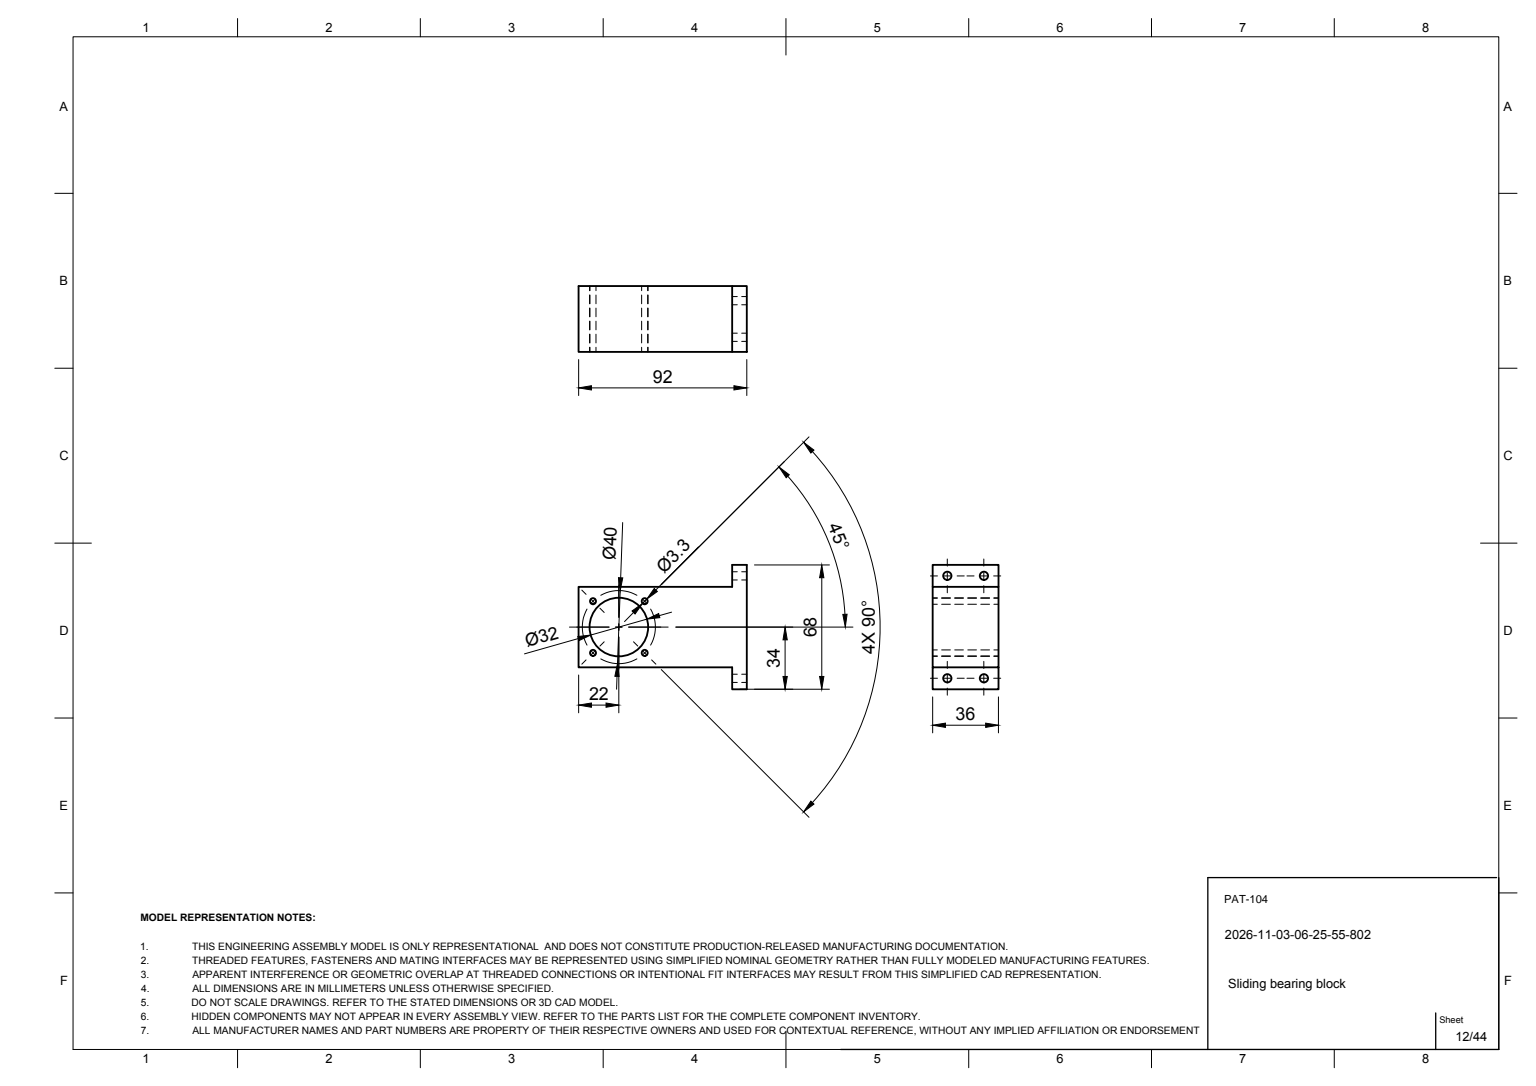
ISO-10303-21;
HEADER;
/* Generated by software containing ST-Developer
 * from STEP Tools, Inc. (www.steptools.com) 
 */

FILE_DESCRIPTION(
/* description */ ('Timing belt drive module 2 mm Pitch Timing 20T-40T'),

/* implementation_level */ '2;1');

FILE_NAME(
/* name */ 'Sliding bearing block.step',
/* time_stamp */ '2026-10-28T03:25:12-07:00',
/* author */ (''),
/* organization */ (''),
/* preprocessor_version */ 'ST-DEVELOPER v20.2',
/* originating_system */ 'Autodesk Translation Framework v15.17.0.0',
/* authorisation */ '');

FILE_SCHEMA (('AUTOMOTIVE_DESIGN { 1 0 10303 214 3 1 1 }'));
ENDSEC;

DATA;
#10=MECHANICAL_DESIGN_GEOMETRIC_PRESENTATION_REPRESENTATION('',(#531),#17830);
#445=SHAPE_REPRESENTATION_RELATIONSHIP('SRR','None',#18015,#488);
#488=ADVANCED_BREP_SHAPE_REPRESENTATION('',(#589),#17790);
#531=STYLED_ITEM('',(#18317),#589);
#589=MANIFOLD_SOLID_BREP('Body1',#8988);
#673=FACE_BOUND('',#1620,.T.);
#674=FACE_BOUND('',#1621,.T.);
#675=FACE_BOUND('',#1623,.T.);
#676=FACE_BOUND('',#1624,.T.);
#677=FACE_BOUND('',#1628,.T.);
#678=FACE_BOUND('',#1629,.T.);
#679=FACE_BOUND('',#1630,.T.);
#680=FACE_BOUND('',#1631,.T.);
#681=FACE_BOUND('',#1632,.T.);
#682=FACE_BOUND('',#1635,.T.);
#683=FACE_BOUND('',#1636,.T.);
#684=FACE_BOUND('',#1637,.T.);
#685=FACE_BOUND('',#1638,.T.);
#686=FACE_BOUND('',#1639,.T.);
#687=FACE_BOUND('',#1643,.T.);
#688=FACE_BOUND('',#1644,.T.);
#689=FACE_BOUND('',#1645,.T.);
#690=FACE_BOUND('',#1646,.T.);
#821=PLANE('',#9734);
#822=PLANE('',#9735);
#823=PLANE('',#9736);
#824=PLANE('',#9737);
#825=PLANE('',#9738);
#826=PLANE('',#9739);
#827=PLANE('',#9740);
#828=PLANE('',#9741);
#829=PLANE('',#9742);
#830=PLANE('',#9743);
#1053=FACE_OUTER_BOUND('',#1610,.T.);
#1054=FACE_OUTER_BOUND('',#1611,.T.);
#1055=FACE_OUTER_BOUND('',#1612,.T.);
#1056=FACE_OUTER_BOUND('',#1613,.T.);
#1057=FACE_OUTER_BOUND('',#1614,.T.);
#1058=FACE_OUTER_BOUND('',#1615,.T.);
#1059=FACE_OUTER_BOUND('',#1616,.T.);
#1060=FACE_OUTER_BOUND('',#1617,.T.);
#1061=FACE_OUTER_BOUND('',#1618,.T.);
#1062=FACE_OUTER_BOUND('',#1619,.T.);
#1063=FACE_OUTER_BOUND('',#1622,.T.);
#1064=FACE_OUTER_BOUND('',#1625,.T.);
#1065=FACE_OUTER_BOUND('',#1626,.T.);
#1066=FACE_OUTER_BOUND('',#1627,.T.);
#1067=FACE_OUTER_BOUND('',#1633,.T.);
#1068=FACE_OUTER_BOUND('',#1634,.T.);
#1069=FACE_OUTER_BOUND('',#1640,.T.);
#1070=FACE_OUTER_BOUND('',#1641,.T.);
#1071=FACE_OUTER_BOUND('',#1642,.T.);
#1610=EDGE_LOOP('',(#6211,#6212,#6213,#6214));
#1611=EDGE_LOOP('',(#6215,#6216,#6217,#6218));
#1612=EDGE_LOOP('',(#6219,#6220,#6221,#6222));
#1613=EDGE_LOOP('',(#6223,#6224,#6225,#6226));
#1614=EDGE_LOOP('',(#6227,#6228,#6229,#6230));
#1615=EDGE_LOOP('',(#6231,#6232,#6233,#6234));
#1616=EDGE_LOOP('',(#6235,#6236,#6237,#6238));
#1617=EDGE_LOOP('',(#6239,#6240,#6241,#6242));
#1618=EDGE_LOOP('',(#6243,#6244,#6245,#6246));
#1619=EDGE_LOOP('',(#6247,#6248,#6249,#6250));
#1620=EDGE_LOOP('',(#6251));
#1621=EDGE_LOOP('',(#6252));
#1622=EDGE_LOOP('',(#6253,#6254,#6255,#6256));
#1623=EDGE_LOOP('',(#6257));
#1624=EDGE_LOOP('',(#6258));
#1625=EDGE_LOOP('',(#6259,#6260,#6261,#6262));
#1626=EDGE_LOOP('',(#6263,#6264,#6265,#6266));
#1627=EDGE_LOOP('',(#6267,#6268,#6269,#6270,#6271,#6272,#6273,#6274));
#1628=EDGE_LOOP('',(#6275));
#1629=EDGE_LOOP('',(#6276));
#1630=EDGE_LOOP('',(#6277));
#1631=EDGE_LOOP('',(#6278));
#1632=EDGE_LOOP('',(#6279));
#1633=EDGE_LOOP('',(#6280,#6281,#6282,#6283));
#1634=EDGE_LOOP('',(#6284,#6285,#6286,#6287,#6288,#6289,#6290,#6291));
#1635=EDGE_LOOP('',(#6292));
#1636=EDGE_LOOP('',(#6293));
#1637=EDGE_LOOP('',(#6294));
#1638=EDGE_LOOP('',(#6295));
#1639=EDGE_LOOP('',(#6296));
#1640=EDGE_LOOP('',(#6297,#6298,#6299,#6300));
#1641=EDGE_LOOP('',(#6301,#6302,#6303,#6304));
#1642=EDGE_LOOP('',(#6305,#6306,#6307,#6308));
#1643=EDGE_LOOP('',(#6309));
#1644=EDGE_LOOP('',(#6310));
#1645=EDGE_LOOP('',(#6311));
#1646=EDGE_LOOP('',(#6312));
#2230=CIRCLE('',#9708,0.165);
#2231=CIRCLE('',#9709,0.165);
#2232=CIRCLE('',#9711,0.165);
#2233=CIRCLE('',#9712,0.165);
#2234=CIRCLE('',#9714,0.164999999999999);
#2235=CIRCLE('',#9715,0.164999999999999);
#2236=CIRCLE('',#9717,0.164999999999999);
#2237=CIRCLE('',#9718,0.164999999999999);
#2238=CIRCLE('',#9720,1.6);
#2239=CIRCLE('',#9721,1.6);
#2240=CIRCLE('',#9723,0.225);
#2241=CIRCLE('',#9724,0.225);
#2242=CIRCLE('',#9726,0.225);
#2243=CIRCLE('',#9727,0.225);
#2244=CIRCLE('',#9729,0.225);
#2245=CIRCLE('',#9730,0.225);
#2246=CIRCLE('',#9732,0.225);
#2247=CIRCLE('',#9733,0.225);
#2919=LINE('',#14343,#3397);
#2920=LINE('',#14349,#3398);
#2921=LINE('',#14355,#3399);
#2922=LINE('',#14361,#3400);
#2923=LINE('',#14367,#3401);
#2924=LINE('',#14373,#3402);
#2925=LINE('',#14379,#3403);
#2926=LINE('',#14385,#3404);
#2927=LINE('',#14391,#3405);
#2928=LINE('',#14396,#3406);
#2929=LINE('',#14398,#3407);
#2930=LINE('',#14400,#3408);
#2931=LINE('',#14401,#3409);
#2932=LINE('',#14405,#3410);
#2933=LINE('',#14407,#3411);
#2934=LINE('',#14409,#3412);
#2935=LINE('',#14410,#3413);
#2936=LINE('',#14413,#3414);
#2937=LINE('',#14415,#3415);
#2938=LINE('',#14416,#3416);
#2939=LINE('',#14419,#3417);
#2940=LINE('',#14421,#3418);
#2941=LINE('',#14422,#3419);
#2942=LINE('',#14425,#3420);
#2943=LINE('',#14427,#3421);
#2944=LINE('',#14428,#3422);
#2945=LINE('',#14429,#3423);
#2946=LINE('',#14432,#3424);
#2947=LINE('',#14433,#3425);
#2948=LINE('',#14436,#3426);
#2949=LINE('',#14437,#3427);
#2950=LINE('',#14438,#3428);
#2951=LINE('',#14440,#3429);
#3397=VECTOR('',#11324,0.165);
#3398=VECTOR('',#11331,0.165);
#3399=VECTOR('',#11338,0.164999999999999);
#3400=VECTOR('',#11345,0.164999999999999);
#3401=VECTOR('',#11352,1.6);
#3402=VECTOR('',#11359,0.225);
#3403=VECTOR('',#11366,0.225);
#3404=VECTOR('',#11373,0.225);
#3405=VECTOR('',#11380,0.225);
#3406=VECTOR('',#11385,1.);
#3407=VECTOR('',#11386,1.);
#3408=VECTOR('',#11387,1.);
#3409=VECTOR('',#11388,1.);
#3410=VECTOR('',#11391,1.);
#3411=VECTOR('',#11392,1.);
#3412=VECTOR('',#11393,1.);
#3413=VECTOR('',#11394,1.);
#3414=VECTOR('',#11397,1.);
#3415=VECTOR('',#11398,1.);
#3416=VECTOR('',#11399,1.);
#3417=VECTOR('',#11402,1.);
#3418=VECTOR('',#11403,1.);
#3419=VECTOR('',#11404,1.);
#3420=VECTOR('',#11407,1.);
#3421=VECTOR('',#11408,1.);
#3422=VECTOR('',#11409,1.);
#3423=VECTOR('',#11410,1.);
#3424=VECTOR('',#11413,1.);
#3425=VECTOR('',#11414,1.);
#3426=VECTOR('',#11417,1.);
#3427=VECTOR('',#11418,1.);
#3428=VECTOR('',#11419,1.);
#3429=VECTOR('',#11422,1.);
#3892=VERTEX_POINT('',#14340);
#3893=VERTEX_POINT('',#14342);
#3894=VERTEX_POINT('',#14346);
#3895=VERTEX_POINT('',#14348);
#3896=VERTEX_POINT('',#14352);
#3897=VERTEX_POINT('',#14354);
#3898=VERTEX_POINT('',#14358);
#3899=VERTEX_POINT('',#14360);
#3900=VERTEX_POINT('',#14364);
#3901=VERTEX_POINT('',#14366);
#3902=VERTEX_POINT('',#14370);
#3903=VERTEX_POINT('',#14372);
#3904=VERTEX_POINT('',#14376);
#3905=VERTEX_POINT('',#14378);
#3906=VERTEX_POINT('',#14382);
#3907=VERTEX_POINT('',#14384);
#3908=VERTEX_POINT('',#14388);
#3909=VERTEX_POINT('',#14390);
#3910=VERTEX_POINT('',#14394);
#3911=VERTEX_POINT('',#14395);
#3912=VERTEX_POINT('',#14397);
#3913=VERTEX_POINT('',#14399);
#3914=VERTEX_POINT('',#14403);
#3915=VERTEX_POINT('',#14404);
#3916=VERTEX_POINT('',#14406);
#3917=VERTEX_POINT('',#14408);
#3918=VERTEX_POINT('',#14412);
#3919=VERTEX_POINT('',#14414);
#3920=VERTEX_POINT('',#14418);
#3921=VERTEX_POINT('',#14420);
#3922=VERTEX_POINT('',#14424);
#3923=VERTEX_POINT('',#14426);
#3924=VERTEX_POINT('',#14431);
#3925=VERTEX_POINT('',#14435);
#4788=EDGE_CURVE('',#3892,#3892,#2230,.T.);
#4789=EDGE_CURVE('',#3892,#3893,#2919,.T.);
#4790=EDGE_CURVE('',#3893,#3893,#2231,.T.);
#4791=EDGE_CURVE('',#3894,#3894,#2232,.T.);
#4792=EDGE_CURVE('',#3894,#3895,#2920,.T.);
#4793=EDGE_CURVE('',#3895,#3895,#2233,.T.);
#4794=EDGE_CURVE('',#3896,#3896,#2234,.T.);
#4795=EDGE_CURVE('',#3896,#3897,#2921,.T.);
#4796=EDGE_CURVE('',#3897,#3897,#2235,.T.);
#4797=EDGE_CURVE('',#3898,#3898,#2236,.T.);
#4798=EDGE_CURVE('',#3898,#3899,#2922,.T.);
#4799=EDGE_CURVE('',#3899,#3899,#2237,.T.);
#4800=EDGE_CURVE('',#3900,#3900,#2238,.T.);
#4801=EDGE_CURVE('',#3900,#3901,#2923,.T.);
#4802=EDGE_CURVE('',#3901,#3901,#2239,.T.);
#4803=EDGE_CURVE('',#3902,#3902,#2240,.T.);
#4804=EDGE_CURVE('',#3902,#3903,#2924,.T.);
#4805=EDGE_CURVE('',#3903,#3903,#2241,.T.);
#4806=EDGE_CURVE('',#3904,#3904,#2242,.T.);
#4807=EDGE_CURVE('',#3904,#3905,#2925,.T.);
#4808=EDGE_CURVE('',#3905,#3905,#2243,.T.);
#4809=EDGE_CURVE('',#3906,#3906,#2244,.T.);
#4810=EDGE_CURVE('',#3906,#3907,#2926,.T.);
#4811=EDGE_CURVE('',#3907,#3907,#2245,.T.);
#4812=EDGE_CURVE('',#3908,#3908,#2246,.T.);
#4813=EDGE_CURVE('',#3908,#3909,#2927,.T.);
#4814=EDGE_CURVE('',#3909,#3909,#2247,.T.);
#4815=EDGE_CURVE('',#3910,#3911,#2928,.T.);
#4816=EDGE_CURVE('',#3912,#3910,#2929,.T.);
#4817=EDGE_CURVE('',#3912,#3913,#2930,.T.);
#4818=EDGE_CURVE('',#3911,#3913,#2931,.T.);
#4819=EDGE_CURVE('',#3914,#3915,#2932,.T.);
#4820=EDGE_CURVE('',#3916,#3914,#2933,.T.);
#4821=EDGE_CURVE('',#3917,#3916,#2934,.T.);
#4822=EDGE_CURVE('',#3915,#3917,#2935,.T.);
#4823=EDGE_CURVE('',#3917,#3918,#2936,.T.);
#4824=EDGE_CURVE('',#3919,#3916,#2937,.T.);
#4825=EDGE_CURVE('',#3918,#3919,#2938,.T.);
#4826=EDGE_CURVE('',#3920,#3912,#2939,.T.);
#4827=EDGE_CURVE('',#3920,#3921,#2940,.T.);
#4828=EDGE_CURVE('',#3913,#3921,#2941,.T.);
#4829=EDGE_CURVE('',#3910,#3922,#2942,.T.);
#4830=EDGE_CURVE('',#3923,#3922,#2943,.T.);
#4831=EDGE_CURVE('',#3915,#3923,#2944,.T.);
#4832=EDGE_CURVE('',#3918,#3920,#2945,.T.);
#4833=EDGE_CURVE('',#3911,#3924,#2946,.T.);
#4834=EDGE_CURVE('',#3922,#3924,#2947,.T.);
#4835=EDGE_CURVE('',#3914,#3925,#2948,.T.);
#4836=EDGE_CURVE('',#3924,#3925,#2949,.T.);
#4837=EDGE_CURVE('',#3921,#3919,#2950,.T.);
#4838=EDGE_CURVE('',#3925,#3923,#2951,.T.);
#6211=ORIENTED_EDGE('',*,*,#4788,.F.);
#6212=ORIENTED_EDGE('',*,*,#4789,.T.);
#6213=ORIENTED_EDGE('',*,*,#4790,.F.);
#6214=ORIENTED_EDGE('',*,*,#4789,.F.);
#6215=ORIENTED_EDGE('',*,*,#4791,.F.);
#6216=ORIENTED_EDGE('',*,*,#4792,.T.);
#6217=ORIENTED_EDGE('',*,*,#4793,.F.);
#6218=ORIENTED_EDGE('',*,*,#4792,.F.);
#6219=ORIENTED_EDGE('',*,*,#4794,.F.);
#6220=ORIENTED_EDGE('',*,*,#4795,.T.);
#6221=ORIENTED_EDGE('',*,*,#4796,.F.);
#6222=ORIENTED_EDGE('',*,*,#4795,.F.);
#6223=ORIENTED_EDGE('',*,*,#4797,.F.);
#6224=ORIENTED_EDGE('',*,*,#4798,.T.);
#6225=ORIENTED_EDGE('',*,*,#4799,.F.);
#6226=ORIENTED_EDGE('',*,*,#4798,.F.);
#6227=ORIENTED_EDGE('',*,*,#4800,.F.);
#6228=ORIENTED_EDGE('',*,*,#4801,.T.);
#6229=ORIENTED_EDGE('',*,*,#4802,.F.);
#6230=ORIENTED_EDGE('',*,*,#4801,.F.);
#6231=ORIENTED_EDGE('',*,*,#4803,.F.);
#6232=ORIENTED_EDGE('',*,*,#4804,.T.);
#6233=ORIENTED_EDGE('',*,*,#4805,.F.);
#6234=ORIENTED_EDGE('',*,*,#4804,.F.);
#6235=ORIENTED_EDGE('',*,*,#4806,.F.);
#6236=ORIENTED_EDGE('',*,*,#4807,.T.);
#6237=ORIENTED_EDGE('',*,*,#4808,.F.);
#6238=ORIENTED_EDGE('',*,*,#4807,.F.);
#6239=ORIENTED_EDGE('',*,*,#4809,.F.);
#6240=ORIENTED_EDGE('',*,*,#4810,.T.);
#6241=ORIENTED_EDGE('',*,*,#4811,.F.);
#6242=ORIENTED_EDGE('',*,*,#4810,.F.);
#6243=ORIENTED_EDGE('',*,*,#4812,.F.);
#6244=ORIENTED_EDGE('',*,*,#4813,.T.);
#6245=ORIENTED_EDGE('',*,*,#4814,.F.);
#6246=ORIENTED_EDGE('',*,*,#4813,.F.);
#6247=ORIENTED_EDGE('',*,*,#4815,.F.);
#6248=ORIENTED_EDGE('',*,*,#4816,.F.);
#6249=ORIENTED_EDGE('',*,*,#4817,.T.);
#6250=ORIENTED_EDGE('',*,*,#4818,.F.);
#6251=ORIENTED_EDGE('',*,*,#4805,.T.);
#6252=ORIENTED_EDGE('',*,*,#4814,.T.);
#6253=ORIENTED_EDGE('',*,*,#4819,.F.);
#6254=ORIENTED_EDGE('',*,*,#4820,.F.);
#6255=ORIENTED_EDGE('',*,*,#4821,.F.);
#6256=ORIENTED_EDGE('',*,*,#4822,.F.);
#6257=ORIENTED_EDGE('',*,*,#4808,.T.);
#6258=ORIENTED_EDGE('',*,*,#4811,.T.);
#6259=ORIENTED_EDGE('',*,*,#4823,.F.);
#6260=ORIENTED_EDGE('',*,*,#4821,.T.);
#6261=ORIENTED_EDGE('',*,*,#4824,.F.);
#6262=ORIENTED_EDGE('',*,*,#4825,.F.);
#6263=ORIENTED_EDGE('',*,*,#4826,.F.);
#6264=ORIENTED_EDGE('',*,*,#4827,.T.);
#6265=ORIENTED_EDGE('',*,*,#4828,.F.);
#6266=ORIENTED_EDGE('',*,*,#4817,.F.);
#6267=ORIENTED_EDGE('',*,*,#4829,.T.);
#6268=ORIENTED_EDGE('',*,*,#4830,.F.);
#6269=ORIENTED_EDGE('',*,*,#4831,.F.);
#6270=ORIENTED_EDGE('',*,*,#4822,.T.);
#6271=ORIENTED_EDGE('',*,*,#4823,.T.);
#6272=ORIENTED_EDGE('',*,*,#4832,.T.);
#6273=ORIENTED_EDGE('',*,*,#4826,.T.);
#6274=ORIENTED_EDGE('',*,*,#4816,.T.);
#6275=ORIENTED_EDGE('',*,*,#4800,.T.);
#6276=ORIENTED_EDGE('',*,*,#4797,.T.);
#6277=ORIENTED_EDGE('',*,*,#4794,.T.);
#6278=ORIENTED_EDGE('',*,*,#4791,.T.);
#6279=ORIENTED_EDGE('',*,*,#4788,.T.);
#6280=ORIENTED_EDGE('',*,*,#4815,.T.);
#6281=ORIENTED_EDGE('',*,*,#4833,.T.);
#6282=ORIENTED_EDGE('',*,*,#4834,.F.);
#6283=ORIENTED_EDGE('',*,*,#4829,.F.);
#6284=ORIENTED_EDGE('',*,*,#4835,.T.);
#6285=ORIENTED_EDGE('',*,*,#4836,.F.);
#6286=ORIENTED_EDGE('',*,*,#4833,.F.);
#6287=ORIENTED_EDGE('',*,*,#4818,.T.);
#6288=ORIENTED_EDGE('',*,*,#4828,.T.);
#6289=ORIENTED_EDGE('',*,*,#4837,.T.);
#6290=ORIENTED_EDGE('',*,*,#4824,.T.);
#6291=ORIENTED_EDGE('',*,*,#4820,.T.);
#6292=ORIENTED_EDGE('',*,*,#4802,.T.);
#6293=ORIENTED_EDGE('',*,*,#4799,.T.);
#6294=ORIENTED_EDGE('',*,*,#4796,.T.);
#6295=ORIENTED_EDGE('',*,*,#4793,.T.);
#6296=ORIENTED_EDGE('',*,*,#4790,.T.);
#6297=ORIENTED_EDGE('',*,*,#4819,.T.);
#6298=ORIENTED_EDGE('',*,*,#4831,.T.);
#6299=ORIENTED_EDGE('',*,*,#4838,.F.);
#6300=ORIENTED_EDGE('',*,*,#4835,.F.);
#6301=ORIENTED_EDGE('',*,*,#4838,.T.);
#6302=ORIENTED_EDGE('',*,*,#4830,.T.);
#6303=ORIENTED_EDGE('',*,*,#4834,.T.);
#6304=ORIENTED_EDGE('',*,*,#4836,.T.);
#6305=ORIENTED_EDGE('',*,*,#4837,.F.);
#6306=ORIENTED_EDGE('',*,*,#4827,.F.);
#6307=ORIENTED_EDGE('',*,*,#4832,.F.);
#6308=ORIENTED_EDGE('',*,*,#4825,.T.);
#6309=ORIENTED_EDGE('',*,*,#4803,.T.);
#6310=ORIENTED_EDGE('',*,*,#4806,.T.);
#6311=ORIENTED_EDGE('',*,*,#4809,.T.);
#6312=ORIENTED_EDGE('',*,*,#4812,.T.);
#8224=CYLINDRICAL_SURFACE('',#9707,0.165);
#8225=CYLINDRICAL_SURFACE('',#9710,0.165);
#8226=CYLINDRICAL_SURFACE('',#9713,0.164999999999999);
#8227=CYLINDRICAL_SURFACE('',#9716,0.164999999999999);
#8228=CYLINDRICAL_SURFACE('',#9719,1.6);
#8229=CYLINDRICAL_SURFACE('',#9722,0.225);
#8230=CYLINDRICAL_SURFACE('',#9725,0.225);
#8231=CYLINDRICAL_SURFACE('',#9728,0.225);
#8232=CYLINDRICAL_SURFACE('',#9731,0.225);
#8551=ADVANCED_FACE('',(#1053),#8224,.F.);
#8552=ADVANCED_FACE('',(#1054),#8225,.F.);
#8553=ADVANCED_FACE('',(#1055),#8226,.F.);
#8554=ADVANCED_FACE('',(#1056),#8227,.F.);
#8555=ADVANCED_FACE('',(#1057),#8228,.F.);
#8556=ADVANCED_FACE('',(#1058),#8229,.F.);
#8557=ADVANCED_FACE('',(#1059),#8230,.F.);
#8558=ADVANCED_FACE('',(#1060),#8231,.F.);
#8559=ADVANCED_FACE('',(#1061),#8232,.F.);
#8560=ADVANCED_FACE('',(#1062,#673,#674),#821,.T.);
#8561=ADVANCED_FACE('',(#1063,#675,#676),#822,.T.);
#8562=ADVANCED_FACE('',(#1064),#823,.T.);
#8563=ADVANCED_FACE('',(#1065),#824,.T.);
#8564=ADVANCED_FACE('',(#1066,#677,#678,#679,#680,#681),#825,.T.);
#8565=ADVANCED_FACE('',(#1067),#826,.T.);
#8566=ADVANCED_FACE('',(#1068,#682,#683,#684,#685,#686),#827,.T.);
#8567=ADVANCED_FACE('',(#1069),#828,.T.);
#8568=ADVANCED_FACE('',(#1070),#829,.T.);
#8569=ADVANCED_FACE('',(#1071,#687,#688,#689,#690),#830,.F.);
#8988=CLOSED_SHELL('',(#8551,#8552,#8553,#8554,#8555,#8556,#8557,#8558,
#8559,#8560,#8561,#8562,#8563,#8564,#8565,#8566,#8567,#8568,#8569));
#9706=AXIS2_PLACEMENT_3D('',#14338,#11318,#11319);
#9707=AXIS2_PLACEMENT_3D('',#14339,#11320,#11321);
#9708=AXIS2_PLACEMENT_3D('',#14341,#11322,#11323);
#9709=AXIS2_PLACEMENT_3D('',#14344,#11325,#11326);
#9710=AXIS2_PLACEMENT_3D('',#14345,#11327,#11328);
#9711=AXIS2_PLACEMENT_3D('',#14347,#11329,#11330);
#9712=AXIS2_PLACEMENT_3D('',#14350,#11332,#11333);
#9713=AXIS2_PLACEMENT_3D('',#14351,#11334,#11335);
#9714=AXIS2_PLACEMENT_3D('',#14353,#11336,#11337);
#9715=AXIS2_PLACEMENT_3D('',#14356,#11339,#11340);
#9716=AXIS2_PLACEMENT_3D('',#14357,#11341,#11342);
#9717=AXIS2_PLACEMENT_3D('',#14359,#11343,#11344);
#9718=AXIS2_PLACEMENT_3D('',#14362,#11346,#11347);
#9719=AXIS2_PLACEMENT_3D('',#14363,#11348,#11349);
#9720=AXIS2_PLACEMENT_3D('',#14365,#11350,#11351);
#9721=AXIS2_PLACEMENT_3D('',#14368,#11353,#11354);
#9722=AXIS2_PLACEMENT_3D('',#14369,#11355,#11356);
#9723=AXIS2_PLACEMENT_3D('',#14371,#11357,#11358);
#9724=AXIS2_PLACEMENT_3D('',#14374,#11360,#11361);
#9725=AXIS2_PLACEMENT_3D('',#14375,#11362,#11363);
#9726=AXIS2_PLACEMENT_3D('',#14377,#11364,#11365);
#9727=AXIS2_PLACEMENT_3D('',#14380,#11367,#11368);
#9728=AXIS2_PLACEMENT_3D('',#14381,#11369,#11370);
#9729=AXIS2_PLACEMENT_3D('',#14383,#11371,#11372);
#9730=AXIS2_PLACEMENT_3D('',#14386,#11374,#11375);
#9731=AXIS2_PLACEMENT_3D('',#14387,#11376,#11377);
#9732=AXIS2_PLACEMENT_3D('',#14389,#11378,#11379);
#9733=AXIS2_PLACEMENT_3D('',#14392,#11381,#11382);
#9734=AXIS2_PLACEMENT_3D('',#14393,#11383,#11384);
#9735=AXIS2_PLACEMENT_3D('',#14402,#11389,#11390);
#9736=AXIS2_PLACEMENT_3D('',#14411,#11395,#11396);
#9737=AXIS2_PLACEMENT_3D('',#14417,#11400,#11401);
#9738=AXIS2_PLACEMENT_3D('',#14423,#11405,#11406);
#9739=AXIS2_PLACEMENT_3D('',#14430,#11411,#11412);
#9740=AXIS2_PLACEMENT_3D('',#14434,#11415,#11416);
#9741=AXIS2_PLACEMENT_3D('',#14439,#11420,#11421);
#9742=AXIS2_PLACEMENT_3D('',#14441,#11423,#11424);
#9743=AXIS2_PLACEMENT_3D('',#14442,#11425,#11426);
#11318=DIRECTION('axis',(0.,0.,1.));
#11319=DIRECTION('refdir',(1.,0.,0.));
#11320=DIRECTION('center_axis',(0.,1.,0.));
#11321=DIRECTION('ref_axis',(1.,0.,0.));
#11322=DIRECTION('center_axis',(0.,1.,0.));
#11323=DIRECTION('ref_axis',(1.,0.,0.));
#11324=DIRECTION('',(0.,1.,0.));
#11325=DIRECTION('center_axis',(0.,-1.,0.));
#11326=DIRECTION('ref_axis',(1.,0.,0.));
#11327=DIRECTION('center_axis',(0.,1.,0.));
#11328=DIRECTION('ref_axis',(1.,0.,0.));
#11329=DIRECTION('center_axis',(0.,1.,0.));
#11330=DIRECTION('ref_axis',(1.,0.,0.));
#11331=DIRECTION('',(0.,1.,0.));
#11332=DIRECTION('center_axis',(0.,-1.,0.));
#11333=DIRECTION('ref_axis',(1.,0.,0.));
#11334=DIRECTION('center_axis',(0.,1.,0.));
#11335=DIRECTION('ref_axis',(1.,0.,0.));
#11336=DIRECTION('center_axis',(0.,1.,0.));
#11337=DIRECTION('ref_axis',(1.,0.,0.));
#11338=DIRECTION('',(0.,1.,0.));
#11339=DIRECTION('center_axis',(0.,-1.,0.));
#11340=DIRECTION('ref_axis',(1.,0.,0.));
#11341=DIRECTION('center_axis',(0.,1.,0.));
#11342=DIRECTION('ref_axis',(1.,0.,0.));
#11343=DIRECTION('center_axis',(0.,1.,0.));
#11344=DIRECTION('ref_axis',(1.,0.,0.));
#11345=DIRECTION('',(0.,1.,0.));
#11346=DIRECTION('center_axis',(0.,-1.,0.));
#11347=DIRECTION('ref_axis',(1.,0.,0.));
#11348=DIRECTION('center_axis',(0.,1.,0.));
#11349=DIRECTION('ref_axis',(1.,0.,0.));
#11350=DIRECTION('center_axis',(0.,1.,0.));
#11351=DIRECTION('ref_axis',(1.,0.,0.));
#11352=DIRECTION('',(0.,1.,0.));
#11353=DIRECTION('center_axis',(0.,-1.,0.));
#11354=DIRECTION('ref_axis',(1.,0.,0.));
#11355=DIRECTION('center_axis',(0.,0.,1.));
#11356=DIRECTION('ref_axis',(1.,0.,0.));
#11357=DIRECTION('center_axis',(0.,0.,1.));
#11358=DIRECTION('ref_axis',(1.,0.,0.));
#11359=DIRECTION('',(0.,0.,1.));
#11360=DIRECTION('center_axis',(0.,0.,-1.));
#11361=DIRECTION('ref_axis',(1.,0.,0.));
#11362=DIRECTION('center_axis',(0.,0.,1.));
#11363=DIRECTION('ref_axis',(1.,0.,0.));
#11364=DIRECTION('center_axis',(0.,0.,1.));
#11365=DIRECTION('ref_axis',(1.,0.,0.));
#11366=DIRECTION('',(0.,0.,1.));
#11367=DIRECTION('center_axis',(0.,0.,-1.));
#11368=DIRECTION('ref_axis',(1.,0.,0.));
#11369=DIRECTION('center_axis',(0.,0.,1.));
#11370=DIRECTION('ref_axis',(1.,0.,0.));
#11371=DIRECTION('center_axis',(0.,0.,1.));
#11372=DIRECTION('ref_axis',(1.,0.,0.));
#11373=DIRECTION('',(0.,0.,1.));
#11374=DIRECTION('center_axis',(0.,0.,-1.));
#11375=DIRECTION('ref_axis',(1.,0.,0.));
#11376=DIRECTION('center_axis',(0.,0.,1.));
#11377=DIRECTION('ref_axis',(1.,0.,0.));
#11378=DIRECTION('center_axis',(0.,0.,1.));
#11379=DIRECTION('ref_axis',(1.,0.,0.));
#11380=DIRECTION('',(0.,0.,1.));
#11381=DIRECTION('center_axis',(0.,0.,-1.));
#11382=DIRECTION('ref_axis',(1.,0.,0.));
#11383=DIRECTION('center_axis',(0.,0.,1.));
#11384=DIRECTION('ref_axis',(1.,0.,0.));
#11385=DIRECTION('',(0.,1.,0.));
#11386=DIRECTION('',(-1.,0.,0.));
#11387=DIRECTION('',(0.,1.,0.));
#11388=DIRECTION('',(1.,0.,0.));
#11389=DIRECTION('center_axis',(0.,0.,1.));
#11390=DIRECTION('ref_axis',(1.,0.,0.));
#11391=DIRECTION('',(0.,-1.,0.));
#11392=DIRECTION('',(1.,0.,0.));
#11393=DIRECTION('',(0.,1.,0.));
#11394=DIRECTION('',(-1.,0.,0.));
#11395=DIRECTION('center_axis',(-1.,0.,0.));
#11396=DIRECTION('ref_axis',(0.,0.,1.));
#11397=DIRECTION('',(0.,0.,-1.));
#11398=DIRECTION('',(0.,0.,1.));
#11399=DIRECTION('',(0.,1.,0.));
#11400=DIRECTION('center_axis',(1.,0.,0.));
#11401=DIRECTION('ref_axis',(0.,0.,-1.));
#11402=DIRECTION('',(0.,0.,1.));
#11403=DIRECTION('',(0.,1.,0.));
#11404=DIRECTION('',(0.,0.,-1.));
#11405=DIRECTION('center_axis',(0.,-1.,0.));
#11406=DIRECTION('ref_axis',(1.,0.,0.));
#11407=DIRECTION('',(0.,0.,1.));
#11408=DIRECTION('',(1.,0.,0.));
#11409=DIRECTION('',(0.,0.,1.));
#11410=DIRECTION('',(1.,0.,0.));
#11411=DIRECTION('center_axis',(1.,0.,0.));
#11412=DIRECTION('ref_axis',(0.,1.,0.));
#11413=DIRECTION('',(0.,0.,1.));
#11414=DIRECTION('',(0.,1.,0.));
#11415=DIRECTION('center_axis',(0.,1.,0.));
#11416=DIRECTION('ref_axis',(-1.,0.,0.));
#11417=DIRECTION('',(0.,0.,1.));
#11418=DIRECTION('',(-1.,0.,0.));
#11419=DIRECTION('',(-1.,0.,0.));
#11420=DIRECTION('center_axis',(-1.,0.,0.));
#11421=DIRECTION('ref_axis',(0.,-1.,0.));
#11422=DIRECTION('',(0.,-1.,0.));
#11423=DIRECTION('center_axis',(0.,0.,1.));
#11424=DIRECTION('ref_axis',(1.,0.,0.));
#11425=DIRECTION('center_axis',(0.,0.,1.));
#11426=DIRECTION('ref_axis',(1.,0.,0.));
#14338=CARTESIAN_POINT('',(0.,0.,0.));
#14339=CARTESIAN_POINT('Origin',(5.55669646780806,-1.9,5.58578643762691));
#14340=CARTESIAN_POINT('',(5.39169646780806,-1.8,5.58578643762691));
#14341=CARTESIAN_POINT('Origin',(5.55669646780806,-1.8,5.58578643762691));
#14342=CARTESIAN_POINT('',(5.39169646780806,1.8,5.58578643762691));
#14343=CARTESIAN_POINT('',(5.39169646780806,-1.9,5.58578643762691));
#14344=CARTESIAN_POINT('Origin',(5.55669646780806,1.8,5.58578643762691));
#14345=CARTESIAN_POINT('Origin',(5.55669646780806,-1.9,8.4142135623731));
#14346=CARTESIAN_POINT('',(5.39169646780806,-1.8,8.4142135623731));
#14347=CARTESIAN_POINT('Origin',(5.55669646780806,-1.8,8.4142135623731));
#14348=CARTESIAN_POINT('',(5.39169646780806,1.8,8.4142135623731));
#14349=CARTESIAN_POINT('',(5.39169646780806,-1.9,8.4142135623731));
#14350=CARTESIAN_POINT('Origin',(5.55669646780806,1.8,8.4142135623731));
#14351=CARTESIAN_POINT('Origin',(8.38512359255425,-1.9,8.4142135623731));
#14352=CARTESIAN_POINT('',(8.22012359255425,-1.8,8.4142135623731));
#14353=CARTESIAN_POINT('Origin',(8.38512359255425,-1.8,8.4142135623731));
#14354=CARTESIAN_POINT('',(8.22012359255425,1.8,8.4142135623731));
#14355=CARTESIAN_POINT('',(8.22012359255425,-1.9,8.4142135623731));
#14356=CARTESIAN_POINT('Origin',(8.38512359255425,1.8,8.4142135623731));
#14357=CARTESIAN_POINT('Origin',(8.38512359255425,-1.9,5.58578643762691));
#14358=CARTESIAN_POINT('',(8.22012359255425,-1.8,5.58578643762691));
#14359=CARTESIAN_POINT('Origin',(8.38512359255425,-1.8,5.58578643762691));
#14360=CARTESIAN_POINT('',(8.22012359255425,1.8,5.58578643762691));
#14361=CARTESIAN_POINT('',(8.22012359255425,-1.9,5.58578643762691));
#14362=CARTESIAN_POINT('Origin',(8.38512359255425,1.8,5.58578643762691));
#14363=CARTESIAN_POINT('Origin',(6.97091003018116,-1.9,7.));
#14364=CARTESIAN_POINT('',(5.37091003018116,-1.8,7.));
#14365=CARTESIAN_POINT('Origin',(6.97091003018116,-1.8,7.));
#14366=CARTESIAN_POINT('',(5.37091003018116,1.8,7.));
#14367=CARTESIAN_POINT('',(5.37091003018116,-1.9,7.));
#14368=CARTESIAN_POINT('Origin',(6.97091003018116,1.8,7.));
#14369=CARTESIAN_POINT('Origin',(9.77091003018116,-1.,-0.1));
#14370=CARTESIAN_POINT('',(9.54591003018116,-1.,0.));
#14371=CARTESIAN_POINT('Origin',(9.77091003018116,-1.,0.));
#14372=CARTESIAN_POINT('',(9.54591003018116,-1.,0.8));
#14373=CARTESIAN_POINT('',(9.54591003018116,-1.,-0.1));
#14374=CARTESIAN_POINT('Origin',(9.77091003018116,-1.,0.8));
#14375=CARTESIAN_POINT('Origin',(4.17091003018116,1.,-0.1));
#14376=CARTESIAN_POINT('',(3.94591003018116,1.,0.));
#14377=CARTESIAN_POINT('Origin',(4.17091003018116,1.,0.));
#14378=CARTESIAN_POINT('',(3.94591003018116,1.,0.8));
#14379=CARTESIAN_POINT('',(3.94591003018116,1.,-0.1));
#14380=CARTESIAN_POINT('Origin',(4.17091003018116,1.,0.8));
#14381=CARTESIAN_POINT('Origin',(4.17091003018116,-1.,-0.1));
#14382=CARTESIAN_POINT('',(3.94591003018116,-1.,0.));
#14383=CARTESIAN_POINT('Origin',(4.17091003018116,-1.,0.));
#14384=CARTESIAN_POINT('',(3.94591003018116,-1.,0.8));
#14385=CARTESIAN_POINT('',(3.94591003018116,-1.,-0.1));
#14386=CARTESIAN_POINT('Origin',(4.17091003018116,-1.,0.8));
#14387=CARTESIAN_POINT('Origin',(9.77091003018116,1.,-0.1));
#14388=CARTESIAN_POINT('',(9.54591003018116,1.,0.));
#14389=CARTESIAN_POINT('Origin',(9.77091003018116,1.,0.));
#14390=CARTESIAN_POINT('',(9.54591003018116,1.,0.8));
#14391=CARTESIAN_POINT('',(9.54591003018116,1.,-0.1));
#14392=CARTESIAN_POINT('Origin',(9.77091003018116,1.,0.8));
#14393=CARTESIAN_POINT('Origin',(3.57091003018116,-1.8,0.8));
#14394=CARTESIAN_POINT('',(9.17091003018116,-1.8,0.8));
#14395=CARTESIAN_POINT('',(9.17091003018116,1.8,0.8));
#14396=CARTESIAN_POINT('',(9.17091003018116,-1.8,0.8));
#14397=CARTESIAN_POINT('',(10.3709100301812,-1.8,0.8));
#14398=CARTESIAN_POINT('',(10.3709100301812,-1.8,0.8));
#14399=CARTESIAN_POINT('',(10.3709100301812,1.8,0.8));
#14400=CARTESIAN_POINT('',(10.3709100301812,-1.8,0.8));
#14401=CARTESIAN_POINT('',(10.3709100301812,1.8,0.8));
#14402=CARTESIAN_POINT('Origin',(3.57091003018116,-1.8,0.8));
#14403=CARTESIAN_POINT('',(4.77091003018116,1.8,0.8));
#14404=CARTESIAN_POINT('',(4.77091003018116,-1.8,0.8));
#14405=CARTESIAN_POINT('',(4.77091003018116,0.,0.8));
#14406=CARTESIAN_POINT('',(3.57091003018116,1.8,0.8));
#14407=CARTESIAN_POINT('',(10.3709100301812,1.8,0.8));
#14408=CARTESIAN_POINT('',(3.57091003018116,-1.8,0.8));
#14409=CARTESIAN_POINT('',(3.57091003018116,-1.8,0.8));
#14410=CARTESIAN_POINT('',(10.3709100301812,-1.8,0.8));
#14411=CARTESIAN_POINT('Origin',(3.57091003018116,-1.8,0.));
#14412=CARTESIAN_POINT('',(3.57091003018116,-1.8,0.));
#14413=CARTESIAN_POINT('',(3.57091003018116,-1.8,0.8));
#14414=CARTESIAN_POINT('',(3.57091003018116,1.8,0.));
#14415=CARTESIAN_POINT('',(3.57091003018116,1.8,0.8));
#14416=CARTESIAN_POINT('',(3.57091003018116,-1.8,0.));
#14417=CARTESIAN_POINT('Origin',(10.3709100301812,-1.8,0.8));
#14418=CARTESIAN_POINT('',(10.3709100301812,-1.8,0.));
#14419=CARTESIAN_POINT('',(10.3709100301812,-1.8,0.));
#14420=CARTESIAN_POINT('',(10.3709100301812,1.8,0.));
#14421=CARTESIAN_POINT('',(10.3709100301812,-1.8,0.));
#14422=CARTESIAN_POINT('',(10.3709100301812,1.8,0.));
#14423=CARTESIAN_POINT('Origin',(4.77091003018116,-1.8,0.));
#14424=CARTESIAN_POINT('',(9.17091003018116,-1.8,9.2));
#14425=CARTESIAN_POINT('',(9.17091003018116,-1.8,0.));
#14426=CARTESIAN_POINT('',(4.77091003018116,-1.8,9.2));
#14427=CARTESIAN_POINT('',(4.77091003018116,-1.8,9.2));
#14428=CARTESIAN_POINT('',(4.77091003018116,-1.8,0.));
#14429=CARTESIAN_POINT('',(3.57091003018116,-1.8,0.));
#14430=CARTESIAN_POINT('Origin',(9.17091003018116,-1.8,0.));
#14431=CARTESIAN_POINT('',(9.17091003018116,1.8,9.2));
#14432=CARTESIAN_POINT('',(9.17091003018116,1.8,0.));
#14433=CARTESIAN_POINT('',(9.17091003018116,-1.8,9.2));
#14434=CARTESIAN_POINT('Origin',(9.17091003018116,1.8,0.));
#14435=CARTESIAN_POINT('',(4.77091003018116,1.8,9.2));
#14436=CARTESIAN_POINT('',(4.77091003018116,1.8,0.));
#14437=CARTESIAN_POINT('',(9.17091003018116,1.8,9.2));
#14438=CARTESIAN_POINT('',(3.57091003018116,1.8,0.));
#14439=CARTESIAN_POINT('Origin',(4.77091003018116,1.8,0.));
#14440=CARTESIAN_POINT('',(4.77091003018116,1.8,9.2));
#14441=CARTESIAN_POINT('Origin',(6.97091003018116,0.,9.2));
#14442=CARTESIAN_POINT('Origin',(6.97091003018116,0.,0.));
#17740=UNCERTAINTY_MEASURE_WITH_UNIT(LENGTH_MEASURE(0.001),#17831,
'DISTANCE_ACCURACY_VALUE',
'Maximum model space distance between geometric entities at asserted c
onnectivities');
#17780=UNCERTAINTY_MEASURE_WITH_UNIT(LENGTH_MEASURE(0.001),#17831,
'DISTANCE_ACCURACY_VALUE',
'Maximum model space distance between geometric entities at asserted c
onnectivities');
#17790=(
GEOMETRIC_REPRESENTATION_CONTEXT(3)
GLOBAL_UNCERTAINTY_ASSIGNED_CONTEXT((#17740))
GLOBAL_UNIT_ASSIGNED_CONTEXT((#17831,#17833,#17834))
REPRESENTATION_CONTEXT('','3D')
);
#17830=(
GEOMETRIC_REPRESENTATION_CONTEXT(3)
GLOBAL_UNCERTAINTY_ASSIGNED_CONTEXT((#17780))
GLOBAL_UNIT_ASSIGNED_CONTEXT((#17831,#17833,#17834))
REPRESENTATION_CONTEXT('','3D')
);
#17831=(
LENGTH_UNIT()
NAMED_UNIT(*)
SI_UNIT(.CENTI.,.METRE.)
);
#17833=(
NAMED_UNIT(*)
PLANE_ANGLE_UNIT()
SI_UNIT($,.RADIAN.)
);
#17834=(
NAMED_UNIT(*)
SI_UNIT($,.STERADIAN.)
SOLID_ANGLE_UNIT()
);
#17844=SHAPE_DEFINITION_REPRESENTATION(#17893,#18015);
#17893=PRODUCT_DEFINITION_SHAPE('',$,#18065);
#18015=SHAPE_REPRESENTATION('',(#9706),#17790);
#18055=PRODUCT_DEFINITION_CONTEXT('part definition',#18204,'design');
#18065=PRODUCT_DEFINITION('Sliding bearing block',
'Sliding bearing block',#18114,#18055);
#18114=PRODUCT_DEFINITION_FORMATION('',$,#18215);
#18204=APPLICATION_CONTEXT(
'Core Data for Automotive Mechanical Design Process');
#18205=PRODUCT_CONTEXT('part definition',#18204,'mechanical');
#18215=PRODUCT('Sliding bearing block','Sliding bearing block',
'Sliding bearing block',(#18205));
#18311=COLOUR_RGB('Grey',0.48,0.52,0.57);
#18312=FILL_AREA_STYLE_COLOUR('',#18311);
#18313=FILL_AREA_STYLE('',(#18312));
#18314=SURFACE_STYLE_FILL_AREA(#18313);
#18315=SURFACE_SIDE_STYLE('',(#18314));
#18316=SURFACE_STYLE_USAGE(.BOTH.,#18315);
#18317=PRESENTATION_STYLE_ASSIGNMENT((#18316));
ENDSEC;
END-ISO-10303-21;
